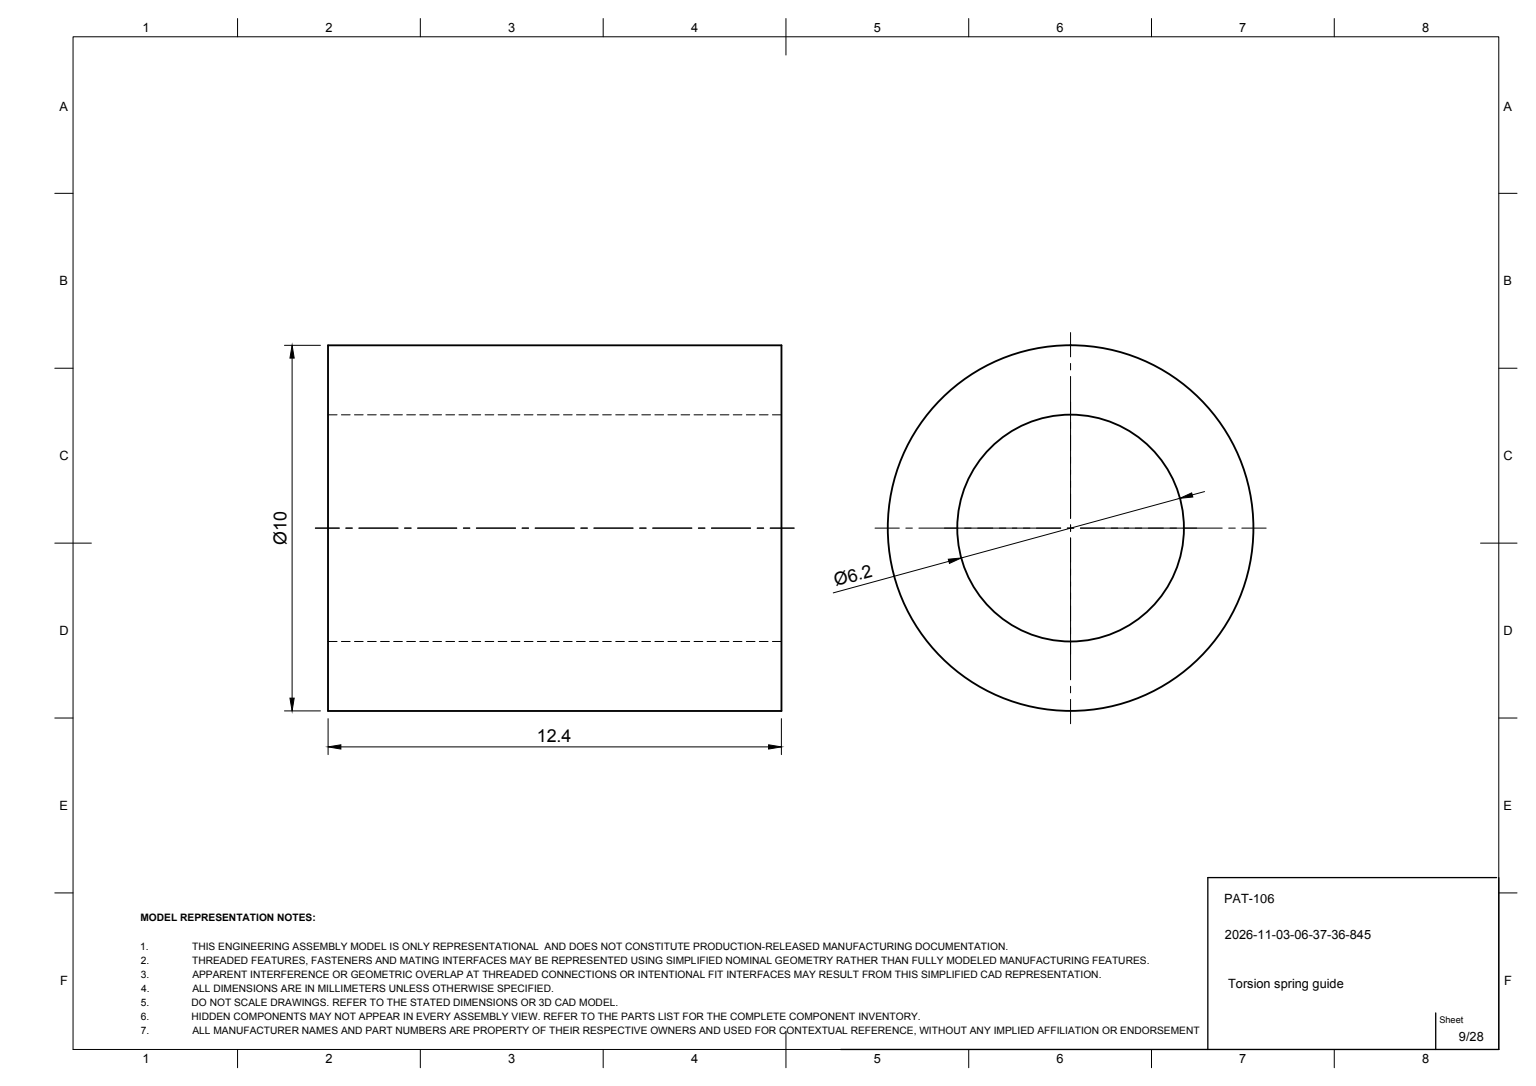
ISO-10303-21;
HEADER;
/* Generated by software containing ST-Developer
 * from STEP Tools, Inc. (www.steptools.com) 
 */

FILE_DESCRIPTION(
/* description */ ('Torsion-spring ratchet demonstrator'),
/* implementation_level */ '2;1');

FILE_NAME(
/* name */ 'Torsion spring guide.step',
/* time_stamp */ '2026-10-29T17:29:17-07:00',
/* author */ (''),
/* organization */ (''),
/* preprocessor_version */ 'ST-DEVELOPER v20.2',
/* originating_system */ 'Autodesk Translation Framework v15.17.0.0',
/* authorisation */ '');

FILE_SCHEMA (('AUTOMOTIVE_DESIGN { 1 0 10303 214 3 1 1 }'));
ENDSEC;

DATA;
#10=MECHANICAL_DESIGN_GEOMETRIC_PRESENTATION_REPRESENTATION('',(#287),#11258);
#239=SHAPE_REPRESENTATION_RELATIONSHIP('SRR','None',#11365,#263);
#263=ADVANCED_BREP_SHAPE_REPRESENTATION('',(#319),#11235);
#287=STYLED_ITEM('',(#11584),#319);
#319=MANIFOLD_SOLID_BREP('Body1',#5158);
#371=FACE_BOUND('',#994,.T.);
#372=FACE_BOUND('',#996,.T.);
#457=PLANE('',#5537);
#458=PLANE('',#5538);
#660=FACE_OUTER_BOUND('',#991,.T.);
#661=FACE_OUTER_BOUND('',#992,.T.);
#662=FACE_OUTER_BOUND('',#993,.T.);
#663=FACE_OUTER_BOUND('',#995,.T.);
#991=EDGE_LOOP('',(#3592,#3593,#3594,#3595));
#992=EDGE_LOOP('',(#3596,#3597,#3598,#3599));
#993=EDGE_LOOP('',(#3600));
#994=EDGE_LOOP('',(#3601));
#995=EDGE_LOOP('',(#3602));
#996=EDGE_LOOP('',(#3603));
#1366=LINE('',#7848,#1749);
#1367=LINE('',#7854,#1750);
#1749=VECTOR('',#6267,0.31);
#1750=VECTOR('',#6274,0.5);
#2125=CIRCLE('',#5532,0.31);
#2126=CIRCLE('',#5533,0.31);
#2127=CIRCLE('',#5535,0.5);
#2128=CIRCLE('',#5536,0.5);
#2385=VERTEX_POINT('',#7845);
#2386=VERTEX_POINT('',#7847);
#2387=VERTEX_POINT('',#7851);
#2388=VERTEX_POINT('',#7853);
#2856=EDGE_CURVE('',#2385,#2385,#2125,.T.);
#2857=EDGE_CURVE('',#2385,#2386,#1366,.T.);
#2858=EDGE_CURVE('',#2386,#2386,#2126,.T.);
#2859=EDGE_CURVE('',#2387,#2387,#2127,.T.);
#2860=EDGE_CURVE('',#2387,#2388,#1367,.T.);
#2861=EDGE_CURVE('',#2388,#2388,#2128,.T.);
#3592=ORIENTED_EDGE('',*,*,#2856,.F.);
#3593=ORIENTED_EDGE('',*,*,#2857,.T.);
#3594=ORIENTED_EDGE('',*,*,#2858,.T.);
#3595=ORIENTED_EDGE('',*,*,#2857,.F.);
#3596=ORIENTED_EDGE('',*,*,#2859,.F.);
#3597=ORIENTED_EDGE('',*,*,#2860,.T.);
#3598=ORIENTED_EDGE('',*,*,#2861,.T.);
#3599=ORIENTED_EDGE('',*,*,#2860,.F.);
#3600=ORIENTED_EDGE('',*,*,#2859,.T.);
#3601=ORIENTED_EDGE('',*,*,#2856,.T.);
#3602=ORIENTED_EDGE('',*,*,#2861,.F.);
#3603=ORIENTED_EDGE('',*,*,#2858,.F.);
#4781=CYLINDRICAL_SURFACE('',#5531,0.31);
#4782=CYLINDRICAL_SURFACE('',#5534,0.5);
#4886=ADVANCED_FACE('',(#660),#4781,.F.);
#4887=ADVANCED_FACE('',(#661),#4782,.T.);
#4888=ADVANCED_FACE('',(#662,#371),#457,.T.);
#4889=ADVANCED_FACE('',(#663,#372),#458,.F.);
#5158=CLOSED_SHELL('',(#4886,#4887,#4888,#4889));
#5530=AXIS2_PLACEMENT_3D('',#7843,#6261,#6262);
#5531=AXIS2_PLACEMENT_3D('',#7844,#6263,#6264);
#5532=AXIS2_PLACEMENT_3D('',#7846,#6265,#6266);
#5533=AXIS2_PLACEMENT_3D('',#7849,#6268,#6269);
#5534=AXIS2_PLACEMENT_3D('',#7850,#6270,#6271);
#5535=AXIS2_PLACEMENT_3D('',#7852,#6272,#6273);
#5536=AXIS2_PLACEMENT_3D('',#7855,#6275,#6276);
#5537=AXIS2_PLACEMENT_3D('',#7856,#6277,#6278);
#5538=AXIS2_PLACEMENT_3D('',#7857,#6279,#6280);
#6261=DIRECTION('axis',(0.,0.,1.));
#6262=DIRECTION('refdir',(1.,0.,0.));
#6263=DIRECTION('center_axis',(0.,0.,1.));
#6264=DIRECTION('ref_axis',(1.,0.,0.));
#6265=DIRECTION('center_axis',(0.,0.,-1.));
#6266=DIRECTION('ref_axis',(1.,0.,0.));
#6267=DIRECTION('',(0.,0.,-1.));
#6268=DIRECTION('center_axis',(0.,0.,-1.));
#6269=DIRECTION('ref_axis',(1.,0.,0.));
#6270=DIRECTION('center_axis',(0.,0.,1.));
#6271=DIRECTION('ref_axis',(1.,0.,0.));
#6272=DIRECTION('center_axis',(0.,0.,1.));
#6273=DIRECTION('ref_axis',(1.,0.,0.));
#6274=DIRECTION('',(0.,0.,-1.));
#6275=DIRECTION('center_axis',(0.,0.,1.));
#6276=DIRECTION('ref_axis',(1.,0.,0.));
#6277=DIRECTION('center_axis',(0.,0.,1.));
#6278=DIRECTION('ref_axis',(1.,0.,0.));
#6279=DIRECTION('center_axis',(0.,0.,1.));
#6280=DIRECTION('ref_axis',(1.,0.,0.));
#7843=CARTESIAN_POINT('',(0.,0.,0.));
#7844=CARTESIAN_POINT('Origin',(6.5,-3.47,5.4));
#7845=CARTESIAN_POINT('',(6.19,-3.47,6.64));
#7846=CARTESIAN_POINT('Origin',(6.5,-3.47,6.64));
#7847=CARTESIAN_POINT('',(6.19,-3.47,5.4));
#7848=CARTESIAN_POINT('',(6.19,-3.47,5.4));
#7849=CARTESIAN_POINT('Origin',(6.5,-3.47,5.4));
#7850=CARTESIAN_POINT('Origin',(6.5,-3.47,5.4));
#7851=CARTESIAN_POINT('',(6.,-3.47,6.64));
#7852=CARTESIAN_POINT('Origin',(6.5,-3.47,6.64));
#7853=CARTESIAN_POINT('',(6.,-3.47,5.4));
#7854=CARTESIAN_POINT('',(6.,-3.47,5.4));
#7855=CARTESIAN_POINT('Origin',(6.5,-3.47,5.4));
#7856=CARTESIAN_POINT('Origin',(6.5,-3.47,6.64));
#7857=CARTESIAN_POINT('Origin',(6.5,-3.47,5.4));
#11205=UNCERTAINTY_MEASURE_WITH_UNIT(LENGTH_MEASURE(0.001),#11259,
'DISTANCE_ACCURACY_VALUE',
'Maximum model space distance between geometric entities at asserted c
onnectivities');
#11228=UNCERTAINTY_MEASURE_WITH_UNIT(LENGTH_MEASURE(0.001),#11259,
'DISTANCE_ACCURACY_VALUE',
'Maximum model space distance between geometric entities at asserted c
onnectivities');
#11235=(
GEOMETRIC_REPRESENTATION_CONTEXT(3)
GLOBAL_UNCERTAINTY_ASSIGNED_CONTEXT((#11205))
GLOBAL_UNIT_ASSIGNED_CONTEXT((#11259,#11261,#11262))
REPRESENTATION_CONTEXT('','3D')
);
#11258=(
GEOMETRIC_REPRESENTATION_CONTEXT(3)
GLOBAL_UNCERTAINTY_ASSIGNED_CONTEXT((#11228))
GLOBAL_UNIT_ASSIGNED_CONTEXT((#11259,#11261,#11262))
REPRESENTATION_CONTEXT('','3D')
);
#11259=(
LENGTH_UNIT()
NAMED_UNIT(*)
SI_UNIT(.CENTI.,.METRE.)
);
#11261=(
NAMED_UNIT(*)
PLANE_ANGLE_UNIT()
SI_UNIT($,.RADIAN.)
);
#11262=(
NAMED_UNIT(*)
SI_UNIT($,.STERADIAN.)
SOLID_ANGLE_UNIT()
);
#11269=SHAPE_DEFINITION_REPRESENTATION(#11298,#11365);
#11298=PRODUCT_DEFINITION_SHAPE('',$,#11395);
#11365=SHAPE_REPRESENTATION('',(#5530),#11235);
#11388=PRODUCT_DEFINITION_CONTEXT('part definition',#11477,'design');
#11395=PRODUCT_DEFINITION('Torsion spring guide','Torsion spring guide',
#11424,#11388);
#11424=PRODUCT_DEFINITION_FORMATION('',$,#11485);
#11477=APPLICATION_CONTEXT(
'Core Data for Automotive Mechanical Design Process');
#11478=PRODUCT_CONTEXT('part definition',#11477,'mechanical');
#11485=PRODUCT('Torsion spring guide','Torsion spring guide',
'Torsion spring guide',(#11478));
#11578=COLOUR_RGB('Grey',0.48,0.52,0.57);
#11579=FILL_AREA_STYLE_COLOUR('',#11578);
#11580=FILL_AREA_STYLE('',(#11579));
#11581=SURFACE_STYLE_FILL_AREA(#11580);
#11582=SURFACE_SIDE_STYLE('',(#11581));
#11583=SURFACE_STYLE_USAGE(.BOTH.,#11582);
#11584=PRESENTATION_STYLE_ASSIGNMENT((#11583));
ENDSEC;
END-ISO-10303-21;
